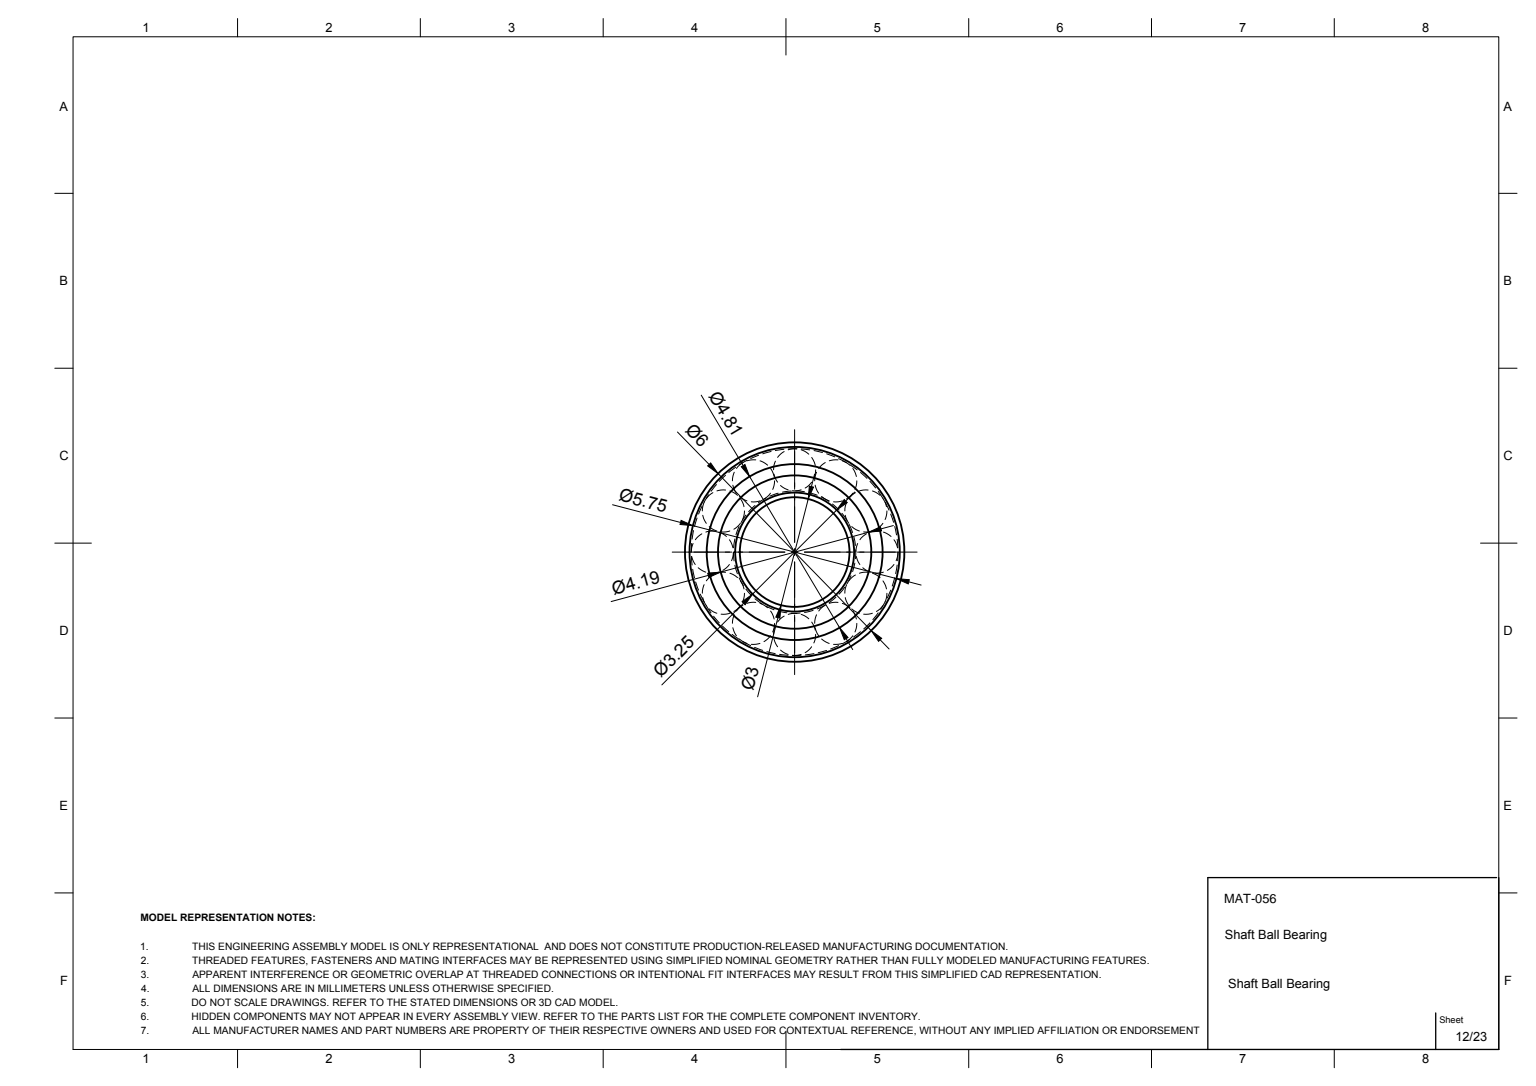
ISO-10303-21;
HEADER;
/* Generated by software containing ST-Developer
 * from STEP Tools, Inc. (www.steptools.com) 
 */

FILE_DESCRIPTION(
/* description */ (''),
/* implementation_level */ '2;1');

FILE_NAME(
/* name */ 'Shaft Ball Bearing.step',
/* time_stamp */ '2026-10-28T16:47:13+01:00',
/* author */ (''),
/* organization */ (''),
/* preprocessor_version */ 'ST-DEVELOPER v20.2',
/* originating_system */ 'Autodesk Translation Framework v15.17.0.0',
/* authorisation */ '');

FILE_SCHEMA (('AUTOMOTIVE_DESIGN { 1 0 10303 214 3 1 1 }'));
ENDSEC;

DATA;
#10=MECHANICAL_DESIGN_GEOMETRIC_PRESENTATION_REPRESENTATION('',(#4589,#4590,#4591,#4592,#4593,#4594,#4595,#4596,#4597,#4598,#4599,#4600,#4601,#4602,#4603,#4604),#459242);
#143=SPHERICAL_SURFACE('',#99208,0.576463888168111);
#144=SPHERICAL_SURFACE('',#99210,0.576463888168111);
#145=SPHERICAL_SURFACE('',#99212,0.576463888168111);
#146=SPHERICAL_SURFACE('',#99214,0.576463888168111);
#147=SPHERICAL_SURFACE('',#99216,0.576463888168111);
#148=SPHERICAL_SURFACE('',#99218,0.576463888168111);
#149=SPHERICAL_SURFACE('',#99220,0.576463888168111);
#150=SPHERICAL_SURFACE('',#99222,0.576463888168111);
#151=SPHERICAL_SURFACE('',#99224,0.576463888168111);
#152=SPHERICAL_SURFACE('',#99226,0.576463888168111);
#153=SPHERICAL_SURFACE('',#99228,0.576463888168111);
#154=SPHERICAL_SURFACE('',#99230,0.576463888168111);
#1862=TOROIDAL_SURFACE('',#99175,2.25,0.576463888168111);
#1863=TOROIDAL_SURFACE('',#99190,2.25,0.57646388816811);
#4416=SHAPE_REPRESENTATION_RELATIONSHIP('SRR','None',#459342,#4437);
#4437=ADVANCED_BREP_SHAPE_REPRESENTATION('',(#4469,#4470,#4471,#4472,#4473,
#4474,#4475,#4476,#4477,#4478,#4479,#4480,#4481,#4482,#4483,#4484),#459231);
#4469=MANIFOLD_SOLID_BREP('Body1',#94647);
#4470=MANIFOLD_SOLID_BREP('Body2',#94648);
#4471=MANIFOLD_SOLID_BREP('Body3',#94649);
#4472=MANIFOLD_SOLID_BREP('Body4',#94650);
#4473=MANIFOLD_SOLID_BREP('Body5',#94651);
#4474=MANIFOLD_SOLID_BREP('Body6',#94652);
#4475=MANIFOLD_SOLID_BREP('Body7',#94653);
#4476=MANIFOLD_SOLID_BREP('Body8',#94654);
#4477=MANIFOLD_SOLID_BREP('Body9',#94655);
#4478=MANIFOLD_SOLID_BREP('Body10',#94656);
#4479=MANIFOLD_SOLID_BREP('Body11',#94657);
#4480=MANIFOLD_SOLID_BREP('Body12',#94658);
#4481=MANIFOLD_SOLID_BREP('Body13',#94659);
#4482=MANIFOLD_SOLID_BREP('Body14',#94660);
#4483=MANIFOLD_SOLID_BREP('Body15',#94661);
#4484=MANIFOLD_SOLID_BREP('Body16',#94662);
#4589=STYLED_ITEM('',(#459526),#4469);
#4590=STYLED_ITEM('',(#459526),#4470);
#4591=STYLED_ITEM('',(#459526),#4471);
#4592=STYLED_ITEM('',(#459526),#4472);
#4593=STYLED_ITEM('',(#459526),#4473);
#4594=STYLED_ITEM('',(#459526),#4474);
#4595=STYLED_ITEM('',(#459526),#4475);
#4596=STYLED_ITEM('',(#459526),#4476);
#4597=STYLED_ITEM('',(#459526),#4477);
#4598=STYLED_ITEM('',(#459526),#4478);
#4599=STYLED_ITEM('',(#459526),#4479);
#4600=STYLED_ITEM('',(#459526),#4480);
#4601=STYLED_ITEM('',(#459526),#4481);
#4602=STYLED_ITEM('',(#459526),#4482);
#4603=STYLED_ITEM('',(#459526),#4483);
#4604=STYLED_ITEM('',(#459526),#4484);
#4884=CONICAL_SURFACE('',#99180,2.875,0.78539816339745);
#4885=CONICAL_SURFACE('',#99186,3.,0.785398163397449);
#4886=CONICAL_SURFACE('',#99194,1.625,0.785398163397448);
#4887=CONICAL_SURFACE('',#99200,1.5,0.785398163397449);
#5213=FACE_BOUND('',#14323,.T.);
#5214=FACE_BOUND('',#14325,.T.);
#5215=FACE_BOUND('',#14333,.T.);
#5216=FACE_BOUND('',#14335,.T.);
#5217=FACE_BOUND('',#14351,.T.);
#5218=FACE_BOUND('',#14353,.T.);
#5219=FACE_BOUND('',#14357,.T.);
#5220=FACE_BOUND('',#14359,.T.);
#5697=PLANE('',#99188);
#5698=PLANE('',#99189);
#5699=PLANE('',#99206);
#5700=PLANE('',#99207);
#5701=PLANE('',#99238);
#5702=PLANE('',#99239);
#5703=PLANE('',#99246);
#5704=PLANE('',#99247);
#8408=FACE_OUTER_BOUND('',#14316,.T.);
#8409=FACE_OUTER_BOUND('',#14317,.T.);
#8410=FACE_OUTER_BOUND('',#14318,.T.);
#8411=FACE_OUTER_BOUND('',#14319,.T.);
#8412=FACE_OUTER_BOUND('',#14320,.T.);
#8413=FACE_OUTER_BOUND('',#14321,.T.);
#8414=FACE_OUTER_BOUND('',#14322,.T.);
#8415=FACE_OUTER_BOUND('',#14324,.T.);
#8416=FACE_OUTER_BOUND('',#14326,.T.);
#8417=FACE_OUTER_BOUND('',#14327,.T.);
#8418=FACE_OUTER_BOUND('',#14328,.T.);
#8419=FACE_OUTER_BOUND('',#14329,.T.);
#8420=FACE_OUTER_BOUND('',#14330,.T.);
#8421=FACE_OUTER_BOUND('',#14331,.T.);
#8422=FACE_OUTER_BOUND('',#14332,.T.);
#8423=FACE_OUTER_BOUND('',#14334,.T.);
#8424=FACE_OUTER_BOUND('',#14336,.T.);
#8425=FACE_OUTER_BOUND('',#14337,.T.);
#8426=FACE_OUTER_BOUND('',#14338,.T.);
#8427=FACE_OUTER_BOUND('',#14339,.T.);
#8428=FACE_OUTER_BOUND('',#14340,.T.);
#8429=FACE_OUTER_BOUND('',#14341,.T.);
#8430=FACE_OUTER_BOUND('',#14342,.T.);
#8431=FACE_OUTER_BOUND('',#14343,.T.);
#8432=FACE_OUTER_BOUND('',#14344,.T.);
#8433=FACE_OUTER_BOUND('',#14345,.T.);
#8434=FACE_OUTER_BOUND('',#14346,.T.);
#8435=FACE_OUTER_BOUND('',#14347,.T.);
#8436=FACE_OUTER_BOUND('',#14348,.T.);
#8437=FACE_OUTER_BOUND('',#14349,.T.);
#8438=FACE_OUTER_BOUND('',#14350,.T.);
#8439=FACE_OUTER_BOUND('',#14352,.T.);
#8440=FACE_OUTER_BOUND('',#14354,.T.);
#8441=FACE_OUTER_BOUND('',#14355,.T.);
#8442=FACE_OUTER_BOUND('',#14356,.T.);
#8443=FACE_OUTER_BOUND('',#14358,.T.);
#14316=EDGE_LOOP('',(#69274,#69275,#69276,#69277));
#14317=EDGE_LOOP('',(#69278,#69279,#69280,#69281));
#14318=EDGE_LOOP('',(#69282,#69283,#69284,#69285));
#14319=EDGE_LOOP('',(#69286,#69287,#69288,#69289));
#14320=EDGE_LOOP('',(#69290,#69291,#69292,#69293,#69294));
#14321=EDGE_LOOP('',(#69295,#69296,#69297,#69298,#69299));
#14322=EDGE_LOOP('',(#69300));
#14323=EDGE_LOOP('',(#69301));
#14324=EDGE_LOOP('',(#69302));
#14325=EDGE_LOOP('',(#69303));
#14326=EDGE_LOOP('',(#69304,#69305,#69306,#69307));
#14327=EDGE_LOOP('',(#69308,#69309,#69310,#69311));
#14328=EDGE_LOOP('',(#69312,#69313,#69314,#69315,#69316));
#14329=EDGE_LOOP('',(#69317,#69318,#69319,#69320,#69321));
#14330=EDGE_LOOP('',(#69322,#69323,#69324,#69325));
#14331=EDGE_LOOP('',(#69326,#69327,#69328,#69329));
#14332=EDGE_LOOP('',(#69330));
#14333=EDGE_LOOP('',(#69331));
#14334=EDGE_LOOP('',(#69332));
#14335=EDGE_LOOP('',(#69333));
#14336=EDGE_LOOP('',(#69334,#69335));
#14337=EDGE_LOOP('',(#69336,#69337));
#14338=EDGE_LOOP('',(#69338,#69339));
#14339=EDGE_LOOP('',(#69340,#69341));
#14340=EDGE_LOOP('',(#69342,#69343));
#14341=EDGE_LOOP('',(#69344,#69345));
#14342=EDGE_LOOP('',(#69346,#69347));
#14343=EDGE_LOOP('',(#69348,#69349));
#14344=EDGE_LOOP('',(#69350,#69351));
#14345=EDGE_LOOP('',(#69352,#69353));
#14346=EDGE_LOOP('',(#69354,#69355));
#14347=EDGE_LOOP('',(#69356,#69357));
#14348=EDGE_LOOP('',(#69358,#69359,#69360,#69361));
#14349=EDGE_LOOP('',(#69362,#69363,#69364,#69365));
#14350=EDGE_LOOP('',(#69366));
#14351=EDGE_LOOP('',(#69367));
#14352=EDGE_LOOP('',(#69368));
#14353=EDGE_LOOP('',(#69369));
#14354=EDGE_LOOP('',(#69370,#69371,#69372,#69373));
#14355=EDGE_LOOP('',(#69374,#69375,#69376,#69377));
#14356=EDGE_LOOP('',(#69378));
#14357=EDGE_LOOP('',(#69379));
#14358=EDGE_LOOP('',(#69380));
#14359=EDGE_LOOP('',(#69381));
#20534=CIRCLE('',#99173,2.40384615384615);
#20535=CIRCLE('',#99174,2.40384615384615);
#20536=CIRCLE('',#99176,2.40384615384615);
#20537=CIRCLE('',#99177,0.576463888168111);
#20538=CIRCLE('',#99179,2.40384615384615);
#20539=CIRCLE('',#99181,3.);
#20540=CIRCLE('',#99182,2.875);
#20541=CIRCLE('',#99184,3.);
#20542=CIRCLE('',#99185,3.);
#20543=CIRCLE('',#99187,2.875);
#20544=CIRCLE('',#99191,2.09615384615385);
#20545=CIRCLE('',#99192,0.57646388816811);
#20546=CIRCLE('',#99193,2.09615384615385);
#20547=CIRCLE('',#99195,1.5);
#20548=CIRCLE('',#99196,1.625);
#20549=CIRCLE('',#99198,1.5);
#20550=CIRCLE('',#99199,1.5);
#20551=CIRCLE('',#99201,1.625);
#20552=CIRCLE('',#99203,2.09615384615385);
#20553=CIRCLE('',#99205,2.09615384615385);
#20554=CIRCLE('',#99209,0.576463888168111);
#20555=CIRCLE('',#99211,0.576463888168111);
#20556=CIRCLE('',#99213,0.576463888168111);
#20557=CIRCLE('',#99215,0.576463888168111);
#20558=CIRCLE('',#99217,0.576463888168111);
#20559=CIRCLE('',#99219,0.576463888168111);
#20560=CIRCLE('',#99221,0.576463888168111);
#20561=CIRCLE('',#99223,0.576463888168111);
#20562=CIRCLE('',#99225,0.576463888168111);
#20563=CIRCLE('',#99227,0.576463888168111);
#20564=CIRCLE('',#99229,0.576463888168111);
#20565=CIRCLE('',#99231,0.576463888168111);
#20566=CIRCLE('',#99233,2.40384615384615);
#20567=CIRCLE('',#99234,2.40384615384615);
#20568=CIRCLE('',#99236,2.09615384615385);
#20569=CIRCLE('',#99237,2.09615384615385);
#20570=CIRCLE('',#99241,2.40384615384615);
#20571=CIRCLE('',#99242,2.40384615384615);
#20572=CIRCLE('',#99244,2.09615384615385);
#20573=CIRCLE('',#99245,2.09615384615385);
#28975=LINE('',#366189,#32777);
#28976=LINE('',#366198,#32778);
#28977=LINE('',#366203,#32779);
#28978=LINE('',#366210,#32780);
#28979=LINE('',#366213,#32781);
#28980=LINE('',#366227,#32782);
#28981=LINE('',#366234,#32783);
#28982=LINE('',#366237,#32784);
#28983=LINE('',#366241,#32785);
#28984=LINE('',#366246,#32786);
#28985=LINE('',#366301,#32787);
#28986=LINE('',#366307,#32788);
#28987=LINE('',#366315,#32789);
#28988=LINE('',#366321,#32790);
#32777=VECTOR('',#116043,2.40384615384615);
#32778=VECTOR('',#116056,2.40384615384615);
#32779=VECTOR('',#116061,2.875);
#32780=VECTOR('',#116070,3.);
#32781=VECTOR('',#116073,3.);
#32782=VECTOR('',#116092,1.625);
#32783=VECTOR('',#116101,1.5);
#32784=VECTOR('',#116104,1.5);
#32785=VECTOR('',#116109,2.09615384615385);
#32786=VECTOR('',#116116,2.09615384615385);
#32787=VECTOR('',#116173,2.40384615384615);
#32788=VECTOR('',#116180,2.09615384615385);
#32789=VECTOR('',#116191,2.40384615384615);
#32790=VECTOR('',#116198,2.09615384615385);
#38293=VERTEX_POINT('',#366186);
#38294=VERTEX_POINT('',#366188);
#38295=VERTEX_POINT('',#366192);
#38296=VERTEX_POINT('',#366196);
#38297=VERTEX_POINT('',#366200);
#38298=VERTEX_POINT('',#366202);
#38299=VERTEX_POINT('',#366206);
#38300=VERTEX_POINT('',#366207);
#38301=VERTEX_POINT('',#366212);
#38302=VERTEX_POINT('',#366218);
#38303=VERTEX_POINT('',#366220);
#38304=VERTEX_POINT('',#366224);
#38305=VERTEX_POINT('',#366226);
#38306=VERTEX_POINT('',#366230);
#38307=VERTEX_POINT('',#366231);
#38308=VERTEX_POINT('',#366236);
#38309=VERTEX_POINT('',#366240);
#38310=VERTEX_POINT('',#366244);
#38311=VERTEX_POINT('',#366250);
#38312=VERTEX_POINT('',#366251);
#38313=VERTEX_POINT('',#366254);
#38314=VERTEX_POINT('',#366255);
#38315=VERTEX_POINT('',#366258);
#38316=VERTEX_POINT('',#366259);
#38317=VERTEX_POINT('',#366262);
#38318=VERTEX_POINT('',#366263);
#38319=VERTEX_POINT('',#366266);
#38320=VERTEX_POINT('',#366267);
#38321=VERTEX_POINT('',#366270);
#38322=VERTEX_POINT('',#366271);
#38323=VERTEX_POINT('',#366274);
#38324=VERTEX_POINT('',#366275);
#38325=VERTEX_POINT('',#366278);
#38326=VERTEX_POINT('',#366279);
#38327=VERTEX_POINT('',#366282);
#38328=VERTEX_POINT('',#366283);
#38329=VERTEX_POINT('',#366286);
#38330=VERTEX_POINT('',#366287);
#38331=VERTEX_POINT('',#366290);
#38332=VERTEX_POINT('',#366291);
#38333=VERTEX_POINT('',#366294);
#38334=VERTEX_POINT('',#366295);
#38335=VERTEX_POINT('',#366298);
#38336=VERTEX_POINT('',#366300);
#38337=VERTEX_POINT('',#366304);
#38338=VERTEX_POINT('',#366306);
#38339=VERTEX_POINT('',#366312);
#38340=VERTEX_POINT('',#366314);
#38341=VERTEX_POINT('',#366318);
#38342=VERTEX_POINT('',#366320);
#49139=EDGE_CURVE('',#38293,#38293,#20534,.T.);
#49140=EDGE_CURVE('',#38293,#38294,#28975,.T.);
#49141=EDGE_CURVE('',#38294,#38294,#20535,.T.);
#49142=EDGE_CURVE('',#38295,#38295,#20536,.T.);
#49143=EDGE_CURVE('',#38295,#38293,#20537,.T.);
#49144=EDGE_CURVE('',#38296,#38296,#20538,.T.);
#49145=EDGE_CURVE('',#38296,#38295,#28976,.T.);
#49146=EDGE_CURVE('',#38297,#38297,#20539,.T.);
#49147=EDGE_CURVE('',#38297,#38298,#28977,.T.);
#49148=EDGE_CURVE('',#38298,#38298,#20540,.T.);
#49149=EDGE_CURVE('',#38299,#38300,#20541,.T.);
#49150=EDGE_CURVE('',#38300,#38299,#20542,.T.);
#49151=EDGE_CURVE('',#38300,#38297,#28978,.T.);
#49152=EDGE_CURVE('',#38299,#38301,#28979,.T.);
#49153=EDGE_CURVE('',#38301,#38301,#20543,.T.);
#49154=EDGE_CURVE('',#38302,#38302,#20544,.T.);
#49155=EDGE_CURVE('',#38302,#38303,#20545,.T.);
#49156=EDGE_CURVE('',#38303,#38303,#20546,.T.);
#49157=EDGE_CURVE('',#38304,#38304,#20547,.T.);
#49158=EDGE_CURVE('',#38304,#38305,#28980,.T.);
#49159=EDGE_CURVE('',#38305,#38305,#20548,.T.);
#49160=EDGE_CURVE('',#38306,#38307,#20549,.T.);
#49161=EDGE_CURVE('',#38307,#38306,#20550,.T.);
#49162=EDGE_CURVE('',#38307,#38304,#28981,.T.);
#49163=EDGE_CURVE('',#38306,#38308,#28982,.T.);
#49164=EDGE_CURVE('',#38308,#38308,#20551,.T.);
#49165=EDGE_CURVE('',#38303,#38309,#28983,.T.);
#49166=EDGE_CURVE('',#38309,#38309,#20552,.T.);
#49167=EDGE_CURVE('',#38310,#38310,#20553,.T.);
#49168=EDGE_CURVE('',#38310,#38302,#28984,.T.);
#49169=EDGE_CURVE('',#38311,#38312,#20554,.T.);
#49170=EDGE_CURVE('',#38313,#38314,#20555,.T.);
#49171=EDGE_CURVE('',#38315,#38316,#20556,.T.);
#49172=EDGE_CURVE('',#38317,#38318,#20557,.T.);
#49173=EDGE_CURVE('',#38319,#38320,#20558,.T.);
#49174=EDGE_CURVE('',#38321,#38322,#20559,.T.);
#49175=EDGE_CURVE('',#38323,#38324,#20560,.T.);
#49176=EDGE_CURVE('',#38325,#38326,#20561,.T.);
#49177=EDGE_CURVE('',#38327,#38328,#20562,.T.);
#49178=EDGE_CURVE('',#38329,#38330,#20563,.T.);
#49179=EDGE_CURVE('',#38331,#38332,#20564,.T.);
#49180=EDGE_CURVE('',#38333,#38334,#20565,.T.);
#49181=EDGE_CURVE('',#38335,#38335,#20566,.T.);
#49182=EDGE_CURVE('',#38335,#38336,#28985,.T.);
#49183=EDGE_CURVE('',#38336,#38336,#20567,.T.);
#49184=EDGE_CURVE('',#38337,#38337,#20568,.T.);
#49185=EDGE_CURVE('',#38337,#38338,#28986,.T.);
#49186=EDGE_CURVE('',#38338,#38338,#20569,.T.);
#49187=EDGE_CURVE('',#38339,#38339,#20570,.T.);
#49188=EDGE_CURVE('',#38339,#38340,#28987,.T.);
#49189=EDGE_CURVE('',#38340,#38340,#20571,.T.);
#49190=EDGE_CURVE('',#38341,#38341,#20572,.T.);
#49191=EDGE_CURVE('',#38341,#38342,#28988,.T.);
#49192=EDGE_CURVE('',#38342,#38342,#20573,.T.);
#69274=ORIENTED_EDGE('',*,*,#49139,.F.);
#69275=ORIENTED_EDGE('',*,*,#49140,.T.);
#69276=ORIENTED_EDGE('',*,*,#49141,.T.);
#69277=ORIENTED_EDGE('',*,*,#49140,.F.);
#69278=ORIENTED_EDGE('',*,*,#49142,.F.);
#69279=ORIENTED_EDGE('',*,*,#49143,.T.);
#69280=ORIENTED_EDGE('',*,*,#49139,.T.);
#69281=ORIENTED_EDGE('',*,*,#49143,.F.);
#69282=ORIENTED_EDGE('',*,*,#49144,.F.);
#69283=ORIENTED_EDGE('',*,*,#49145,.T.);
#69284=ORIENTED_EDGE('',*,*,#49142,.T.);
#69285=ORIENTED_EDGE('',*,*,#49145,.F.);
#69286=ORIENTED_EDGE('',*,*,#49146,.F.);
#69287=ORIENTED_EDGE('',*,*,#49147,.T.);
#69288=ORIENTED_EDGE('',*,*,#49148,.T.);
#69289=ORIENTED_EDGE('',*,*,#49147,.F.);
#69290=ORIENTED_EDGE('',*,*,#49149,.F.);
#69291=ORIENTED_EDGE('',*,*,#49150,.F.);
#69292=ORIENTED_EDGE('',*,*,#49151,.T.);
#69293=ORIENTED_EDGE('',*,*,#49146,.T.);
#69294=ORIENTED_EDGE('',*,*,#49151,.F.);
#69295=ORIENTED_EDGE('',*,*,#49149,.T.);
#69296=ORIENTED_EDGE('',*,*,#49150,.T.);
#69297=ORIENTED_EDGE('',*,*,#49152,.T.);
#69298=ORIENTED_EDGE('',*,*,#49153,.F.);
#69299=ORIENTED_EDGE('',*,*,#49152,.F.);
#69300=ORIENTED_EDGE('',*,*,#49148,.F.);
#69301=ORIENTED_EDGE('',*,*,#49144,.T.);
#69302=ORIENTED_EDGE('',*,*,#49153,.T.);
#69303=ORIENTED_EDGE('',*,*,#49141,.F.);
#69304=ORIENTED_EDGE('',*,*,#49154,.F.);
#69305=ORIENTED_EDGE('',*,*,#49155,.T.);
#69306=ORIENTED_EDGE('',*,*,#49156,.T.);
#69307=ORIENTED_EDGE('',*,*,#49155,.F.);
#69308=ORIENTED_EDGE('',*,*,#49157,.F.);
#69309=ORIENTED_EDGE('',*,*,#49158,.T.);
#69310=ORIENTED_EDGE('',*,*,#49159,.T.);
#69311=ORIENTED_EDGE('',*,*,#49158,.F.);
#69312=ORIENTED_EDGE('',*,*,#49160,.F.);
#69313=ORIENTED_EDGE('',*,*,#49161,.F.);
#69314=ORIENTED_EDGE('',*,*,#49162,.T.);
#69315=ORIENTED_EDGE('',*,*,#49157,.T.);
#69316=ORIENTED_EDGE('',*,*,#49162,.F.);
#69317=ORIENTED_EDGE('',*,*,#49160,.T.);
#69318=ORIENTED_EDGE('',*,*,#49161,.T.);
#69319=ORIENTED_EDGE('',*,*,#49163,.T.);
#69320=ORIENTED_EDGE('',*,*,#49164,.F.);
#69321=ORIENTED_EDGE('',*,*,#49163,.F.);
#69322=ORIENTED_EDGE('',*,*,#49156,.F.);
#69323=ORIENTED_EDGE('',*,*,#49165,.T.);
#69324=ORIENTED_EDGE('',*,*,#49166,.T.);
#69325=ORIENTED_EDGE('',*,*,#49165,.F.);
#69326=ORIENTED_EDGE('',*,*,#49167,.F.);
#69327=ORIENTED_EDGE('',*,*,#49168,.T.);
#69328=ORIENTED_EDGE('',*,*,#49154,.T.);
#69329=ORIENTED_EDGE('',*,*,#49168,.F.);
#69330=ORIENTED_EDGE('',*,*,#49167,.T.);
#69331=ORIENTED_EDGE('',*,*,#49159,.F.);
#69332=ORIENTED_EDGE('',*,*,#49166,.F.);
#69333=ORIENTED_EDGE('',*,*,#49164,.T.);
#69334=ORIENTED_EDGE('',*,*,#49169,.T.);
#69335=ORIENTED_EDGE('',*,*,#49169,.F.);
#69336=ORIENTED_EDGE('',*,*,#49170,.T.);
#69337=ORIENTED_EDGE('',*,*,#49170,.F.);
#69338=ORIENTED_EDGE('',*,*,#49171,.T.);
#69339=ORIENTED_EDGE('',*,*,#49171,.F.);
#69340=ORIENTED_EDGE('',*,*,#49172,.T.);
#69341=ORIENTED_EDGE('',*,*,#49172,.F.);
#69342=ORIENTED_EDGE('',*,*,#49173,.T.);
#69343=ORIENTED_EDGE('',*,*,#49173,.F.);
#69344=ORIENTED_EDGE('',*,*,#49174,.T.);
#69345=ORIENTED_EDGE('',*,*,#49174,.F.);
#69346=ORIENTED_EDGE('',*,*,#49175,.T.);
#69347=ORIENTED_EDGE('',*,*,#49175,.F.);
#69348=ORIENTED_EDGE('',*,*,#49176,.T.);
#69349=ORIENTED_EDGE('',*,*,#49176,.F.);
#69350=ORIENTED_EDGE('',*,*,#49177,.T.);
#69351=ORIENTED_EDGE('',*,*,#49177,.F.);
#69352=ORIENTED_EDGE('',*,*,#49178,.T.);
#69353=ORIENTED_EDGE('',*,*,#49178,.F.);
#69354=ORIENTED_EDGE('',*,*,#49179,.T.);
#69355=ORIENTED_EDGE('',*,*,#49179,.F.);
#69356=ORIENTED_EDGE('',*,*,#49180,.T.);
#69357=ORIENTED_EDGE('',*,*,#49180,.F.);
#69358=ORIENTED_EDGE('',*,*,#49181,.F.);
#69359=ORIENTED_EDGE('',*,*,#49182,.T.);
#69360=ORIENTED_EDGE('',*,*,#49183,.T.);
#69361=ORIENTED_EDGE('',*,*,#49182,.F.);
#69362=ORIENTED_EDGE('',*,*,#49184,.F.);
#69363=ORIENTED_EDGE('',*,*,#49185,.T.);
#69364=ORIENTED_EDGE('',*,*,#49186,.T.);
#69365=ORIENTED_EDGE('',*,*,#49185,.F.);
#69366=ORIENTED_EDGE('',*,*,#49181,.T.);
#69367=ORIENTED_EDGE('',*,*,#49186,.F.);
#69368=ORIENTED_EDGE('',*,*,#49183,.F.);
#69369=ORIENTED_EDGE('',*,*,#49184,.T.);
#69370=ORIENTED_EDGE('',*,*,#49187,.F.);
#69371=ORIENTED_EDGE('',*,*,#49188,.T.);
#69372=ORIENTED_EDGE('',*,*,#49189,.T.);
#69373=ORIENTED_EDGE('',*,*,#49188,.F.);
#69374=ORIENTED_EDGE('',*,*,#49190,.F.);
#69375=ORIENTED_EDGE('',*,*,#49191,.T.);
#69376=ORIENTED_EDGE('',*,*,#49192,.T.);
#69377=ORIENTED_EDGE('',*,*,#49191,.F.);
#69378=ORIENTED_EDGE('',*,*,#49189,.F.);
#69379=ORIENTED_EDGE('',*,*,#49190,.T.);
#69380=ORIENTED_EDGE('',*,*,#49187,.T.);
#69381=ORIENTED_EDGE('',*,*,#49192,.F.);
#87921=CYLINDRICAL_SURFACE('',#99172,2.40384615384615);
#87922=CYLINDRICAL_SURFACE('',#99178,2.40384615384615);
#87923=CYLINDRICAL_SURFACE('',#99183,3.);
#87924=CYLINDRICAL_SURFACE('',#99197,1.5);
#87925=CYLINDRICAL_SURFACE('',#99202,2.09615384615385);
#87926=CYLINDRICAL_SURFACE('',#99204,2.09615384615385);
#87927=CYLINDRICAL_SURFACE('',#99232,2.40384615384615);
#87928=CYLINDRICAL_SURFACE('',#99235,2.09615384615385);
#87929=CYLINDRICAL_SURFACE('',#99240,2.40384615384615);
#87930=CYLINDRICAL_SURFACE('',#99243,2.09615384615385);
#90872=ADVANCED_FACE('',(#8408),#87921,.F.);
#90873=ADVANCED_FACE('',(#8409),#1862,.F.);
#90874=ADVANCED_FACE('',(#8410),#87922,.F.);
#90875=ADVANCED_FACE('',(#8411),#4884,.T.);
#90876=ADVANCED_FACE('',(#8412),#87923,.T.);
#90877=ADVANCED_FACE('',(#8413),#4885,.T.);
#90878=ADVANCED_FACE('',(#8414,#5213),#5697,.F.);
#90879=ADVANCED_FACE('',(#8415,#5214),#5698,.F.);
#90880=ADVANCED_FACE('',(#8416),#1863,.F.);
#90881=ADVANCED_FACE('',(#8417),#4886,.F.);
#90882=ADVANCED_FACE('',(#8418),#87924,.F.);
#90883=ADVANCED_FACE('',(#8419),#4887,.F.);
#90884=ADVANCED_FACE('',(#8420),#87925,.T.);
#90885=ADVANCED_FACE('',(#8421),#87926,.T.);
#90886=ADVANCED_FACE('',(#8422,#5215),#5699,.F.);
#90887=ADVANCED_FACE('',(#8423,#5216),#5700,.F.);
#90888=ADVANCED_FACE('',(#8424),#143,.T.);
#90889=ADVANCED_FACE('',(#8425),#144,.T.);
#90890=ADVANCED_FACE('',(#8426),#145,.T.);
#90891=ADVANCED_FACE('',(#8427),#146,.T.);
#90892=ADVANCED_FACE('',(#8428),#147,.T.);
#90893=ADVANCED_FACE('',(#8429),#148,.T.);
#90894=ADVANCED_FACE('',(#8430),#149,.T.);
#90895=ADVANCED_FACE('',(#8431),#150,.T.);
#90896=ADVANCED_FACE('',(#8432),#151,.T.);
#90897=ADVANCED_FACE('',(#8433),#152,.T.);
#90898=ADVANCED_FACE('',(#8434),#153,.T.);
#90899=ADVANCED_FACE('',(#8435),#154,.T.);
#90900=ADVANCED_FACE('',(#8436),#87927,.T.);
#90901=ADVANCED_FACE('',(#8437),#87928,.F.);
#90902=ADVANCED_FACE('',(#8438,#5217),#5701,.F.);
#90903=ADVANCED_FACE('',(#8439,#5218),#5702,.F.);
#90904=ADVANCED_FACE('',(#8440),#87929,.T.);
#90905=ADVANCED_FACE('',(#8441),#87930,.F.);
#90906=ADVANCED_FACE('',(#8442,#5219),#5703,.F.);
#90907=ADVANCED_FACE('',(#8443,#5220),#5704,.F.);
#94647=CLOSED_SHELL('',(#90872,#90873,#90874,#90875,#90876,#90877,#90878,
#90879));
#94648=CLOSED_SHELL('',(#90880,#90881,#90882,#90883,#90884,#90885,#90886,
#90887));
#94649=CLOSED_SHELL('',(#90888));
#94650=CLOSED_SHELL('',(#90889));
#94651=CLOSED_SHELL('',(#90890));
#94652=CLOSED_SHELL('',(#90891));
#94653=CLOSED_SHELL('',(#90892));
#94654=CLOSED_SHELL('',(#90893));
#94655=CLOSED_SHELL('',(#90894));
#94656=CLOSED_SHELL('',(#90895));
#94657=CLOSED_SHELL('',(#90896));
#94658=CLOSED_SHELL('',(#90897));
#94659=CLOSED_SHELL('',(#90898));
#94660=CLOSED_SHELL('',(#90899));
#94661=CLOSED_SHELL('',(#90900,#90901,#90902,#90903));
#94662=CLOSED_SHELL('',(#90904,#90905,#90906,#90907));
#99171=AXIS2_PLACEMENT_3D('',#366184,#116037,#116038);
#99172=AXIS2_PLACEMENT_3D('',#366185,#116039,#116040);
#99173=AXIS2_PLACEMENT_3D('',#366187,#116041,#116042);
#99174=AXIS2_PLACEMENT_3D('',#366190,#116044,#116045);
#99175=AXIS2_PLACEMENT_3D('',#366191,#116046,#116047);
#99176=AXIS2_PLACEMENT_3D('',#366193,#116048,#116049);
#99177=AXIS2_PLACEMENT_3D('',#366194,#116050,#116051);
#99178=AXIS2_PLACEMENT_3D('',#366195,#116052,#116053);
#99179=AXIS2_PLACEMENT_3D('',#366197,#116054,#116055);
#99180=AXIS2_PLACEMENT_3D('',#366199,#116057,#116058);
#99181=AXIS2_PLACEMENT_3D('',#366201,#116059,#116060);
#99182=AXIS2_PLACEMENT_3D('',#366204,#116062,#116063);
#99183=AXIS2_PLACEMENT_3D('',#366205,#116064,#116065);
#99184=AXIS2_PLACEMENT_3D('',#366208,#116066,#116067);
#99185=AXIS2_PLACEMENT_3D('',#366209,#116068,#116069);
#99186=AXIS2_PLACEMENT_3D('',#366211,#116071,#116072);
#99187=AXIS2_PLACEMENT_3D('',#366214,#116074,#116075);
#99188=AXIS2_PLACEMENT_3D('',#366215,#116076,#116077);
#99189=AXIS2_PLACEMENT_3D('',#366216,#116078,#116079);
#99190=AXIS2_PLACEMENT_3D('',#366217,#116080,#116081);
#99191=AXIS2_PLACEMENT_3D('',#366219,#116082,#116083);
#99192=AXIS2_PLACEMENT_3D('',#366221,#116084,#116085);
#99193=AXIS2_PLACEMENT_3D('',#366222,#116086,#116087);
#99194=AXIS2_PLACEMENT_3D('',#366223,#116088,#116089);
#99195=AXIS2_PLACEMENT_3D('',#366225,#116090,#116091);
#99196=AXIS2_PLACEMENT_3D('',#366228,#116093,#116094);
#99197=AXIS2_PLACEMENT_3D('',#366229,#116095,#116096);
#99198=AXIS2_PLACEMENT_3D('',#366232,#116097,#116098);
#99199=AXIS2_PLACEMENT_3D('',#366233,#116099,#116100);
#99200=AXIS2_PLACEMENT_3D('',#366235,#116102,#116103);
#99201=AXIS2_PLACEMENT_3D('',#366238,#116105,#116106);
#99202=AXIS2_PLACEMENT_3D('',#366239,#116107,#116108);
#99203=AXIS2_PLACEMENT_3D('',#366242,#116110,#116111);
#99204=AXIS2_PLACEMENT_3D('',#366243,#116112,#116113);
#99205=AXIS2_PLACEMENT_3D('',#366245,#116114,#116115);
#99206=AXIS2_PLACEMENT_3D('',#366247,#116117,#116118);
#99207=AXIS2_PLACEMENT_3D('',#366248,#116119,#116120);
#99208=AXIS2_PLACEMENT_3D('',#366249,#116121,#116122);
#99209=AXIS2_PLACEMENT_3D('',#366252,#116123,#116124);
#99210=AXIS2_PLACEMENT_3D('',#366253,#116125,#116126);
#99211=AXIS2_PLACEMENT_3D('',#366256,#116127,#116128);
#99212=AXIS2_PLACEMENT_3D('',#366257,#116129,#116130);
#99213=AXIS2_PLACEMENT_3D('',#366260,#116131,#116132);
#99214=AXIS2_PLACEMENT_3D('',#366261,#116133,#116134);
#99215=AXIS2_PLACEMENT_3D('',#366264,#116135,#116136);
#99216=AXIS2_PLACEMENT_3D('',#366265,#116137,#116138);
#99217=AXIS2_PLACEMENT_3D('',#366268,#116139,#116140);
#99218=AXIS2_PLACEMENT_3D('',#366269,#116141,#116142);
#99219=AXIS2_PLACEMENT_3D('',#366272,#116143,#116144);
#99220=AXIS2_PLACEMENT_3D('',#366273,#116145,#116146);
#99221=AXIS2_PLACEMENT_3D('',#366276,#116147,#116148);
#99222=AXIS2_PLACEMENT_3D('',#366277,#116149,#116150);
#99223=AXIS2_PLACEMENT_3D('',#366280,#116151,#116152);
#99224=AXIS2_PLACEMENT_3D('',#366281,#116153,#116154);
#99225=AXIS2_PLACEMENT_3D('',#366284,#116155,#116156);
#99226=AXIS2_PLACEMENT_3D('',#366285,#116157,#116158);
#99227=AXIS2_PLACEMENT_3D('',#366288,#116159,#116160);
#99228=AXIS2_PLACEMENT_3D('',#366289,#116161,#116162);
#99229=AXIS2_PLACEMENT_3D('',#366292,#116163,#116164);
#99230=AXIS2_PLACEMENT_3D('',#366293,#116165,#116166);
#99231=AXIS2_PLACEMENT_3D('',#366296,#116167,#116168);
#99232=AXIS2_PLACEMENT_3D('',#366297,#116169,#116170);
#99233=AXIS2_PLACEMENT_3D('',#366299,#116171,#116172);
#99234=AXIS2_PLACEMENT_3D('',#366302,#116174,#116175);
#99235=AXIS2_PLACEMENT_3D('',#366303,#116176,#116177);
#99236=AXIS2_PLACEMENT_3D('',#366305,#116178,#116179);
#99237=AXIS2_PLACEMENT_3D('',#366308,#116181,#116182);
#99238=AXIS2_PLACEMENT_3D('',#366309,#116183,#116184);
#99239=AXIS2_PLACEMENT_3D('',#366310,#116185,#116186);
#99240=AXIS2_PLACEMENT_3D('',#366311,#116187,#116188);
#99241=AXIS2_PLACEMENT_3D('',#366313,#116189,#116190);
#99242=AXIS2_PLACEMENT_3D('',#366316,#116192,#116193);
#99243=AXIS2_PLACEMENT_3D('',#366317,#116194,#116195);
#99244=AXIS2_PLACEMENT_3D('',#366319,#116196,#116197);
#99245=AXIS2_PLACEMENT_3D('',#366322,#116199,#116200);
#99246=AXIS2_PLACEMENT_3D('',#366323,#116201,#116202);
#99247=AXIS2_PLACEMENT_3D('',#366324,#116203,#116204);
#116037=DIRECTION('axis',(0.,0.,1.));
#116038=DIRECTION('refdir',(1.,0.,0.));
#116039=DIRECTION('center_axis',(0.,0.,1.));
#116040=DIRECTION('ref_axis',(1.,0.,0.));
#116041=DIRECTION('center_axis',(0.,0.,1.));
#116042=DIRECTION('ref_axis',(1.,0.,0.));
#116043=DIRECTION('',(0.,0.,1.));
#116044=DIRECTION('center_axis',(0.,0.,1.));
#116045=DIRECTION('ref_axis',(1.,0.,0.));
#116046=DIRECTION('center_axis',(0.,0.,1.));
#116047=DIRECTION('ref_axis',(1.,0.,0.));
#116048=DIRECTION('center_axis',(0.,0.,1.));
#116049=DIRECTION('ref_axis',(1.,0.,0.));
#116050=DIRECTION('center_axis',(-1.22464679914735E-16,1.,0.));
#116051=DIRECTION('ref_axis',(-1.,-1.22464679914735E-16,0.));
#116052=DIRECTION('center_axis',(0.,0.,1.));
#116053=DIRECTION('ref_axis',(1.,0.,0.));
#116054=DIRECTION('center_axis',(0.,0.,1.));
#116055=DIRECTION('ref_axis',(1.,0.,0.));
#116056=DIRECTION('',(0.,0.,1.));
#116057=DIRECTION('center_axis',(0.,0.,1.));
#116058=DIRECTION('ref_axis',(1.,0.,0.));
#116059=DIRECTION('center_axis',(0.,0.,1.));
#116060=DIRECTION('ref_axis',(1.,0.,0.));
#116061=DIRECTION('',(0.707106781186549,8.65956056235495E-17,-0.707106781186546));
#116062=DIRECTION('center_axis',(0.,0.,1.));
#116063=DIRECTION('ref_axis',(1.,0.,0.));
#116064=DIRECTION('center_axis',(0.,0.,1.));
#116065=DIRECTION('ref_axis',(1.,0.,0.));
#116066=DIRECTION('center_axis',(0.,0.,1.));
#116067=DIRECTION('ref_axis',(1.,0.,0.));
#116068=DIRECTION('center_axis',(0.,0.,1.));
#116069=DIRECTION('ref_axis',(1.,0.,0.));
#116070=DIRECTION('',(0.,0.,-1.));
#116071=DIRECTION('center_axis',(0.,0.,-1.));
#116072=DIRECTION('ref_axis',(-1.,0.,0.));
#116073=DIRECTION('',(-0.707106781186548,8.65956056235494E-17,0.707106781186547));
#116074=DIRECTION('center_axis',(0.,0.,1.));
#116075=DIRECTION('ref_axis',(1.,0.,0.));
#116076=DIRECTION('center_axis',(0.,0.,1.));
#116077=DIRECTION('ref_axis',(1.,0.,0.));
#116078=DIRECTION('center_axis',(0.,0.,-1.));
#116079=DIRECTION('ref_axis',(-1.,0.,0.));
#116080=DIRECTION('center_axis',(0.,0.,1.));
#116081=DIRECTION('ref_axis',(1.,0.,0.));
#116082=DIRECTION('center_axis',(0.,0.,1.));
#116083=DIRECTION('ref_axis',(1.,0.,0.));
#116084=DIRECTION('center_axis',(-1.22464679914735E-16,1.,0.));
#116085=DIRECTION('ref_axis',(-1.,-1.22464679914735E-16,0.));
#116086=DIRECTION('center_axis',(0.,0.,1.));
#116087=DIRECTION('ref_axis',(1.,0.,0.));
#116088=DIRECTION('center_axis',(0.,0.,1.));
#116089=DIRECTION('ref_axis',(1.,0.,0.));
#116090=DIRECTION('center_axis',(0.,0.,1.));
#116091=DIRECTION('ref_axis',(1.,0.,0.));
#116092=DIRECTION('',(-0.707106781186547,-8.65956056235493E-17,0.707106781186548));
#116093=DIRECTION('center_axis',(0.,0.,1.));
#116094=DIRECTION('ref_axis',(1.,0.,0.));
#116095=DIRECTION('center_axis',(0.,0.,1.));
#116096=DIRECTION('ref_axis',(1.,0.,0.));
#116097=DIRECTION('center_axis',(0.,0.,1.));
#116098=DIRECTION('ref_axis',(1.,0.,0.));
#116099=DIRECTION('center_axis',(0.,0.,1.));
#116100=DIRECTION('ref_axis',(1.,0.,0.));
#116101=DIRECTION('',(0.,0.,1.));
#116102=DIRECTION('center_axis',(0.,0.,-1.));
#116103=DIRECTION('ref_axis',(-1.,0.,0.));
#116104=DIRECTION('',(0.707106781186548,-8.65956056235494E-17,-0.707106781186547));
#116105=DIRECTION('center_axis',(0.,0.,1.));
#116106=DIRECTION('ref_axis',(1.,0.,0.));
#116107=DIRECTION('center_axis',(0.,0.,1.));
#116108=DIRECTION('ref_axis',(1.,0.,0.));
#116109=DIRECTION('',(0.,0.,-1.));
#116110=DIRECTION('center_axis',(0.,0.,1.));
#116111=DIRECTION('ref_axis',(1.,0.,0.));
#116112=DIRECTION('center_axis',(0.,0.,1.));
#116113=DIRECTION('ref_axis',(1.,0.,0.));
#116114=DIRECTION('center_axis',(0.,0.,1.));
#116115=DIRECTION('ref_axis',(1.,0.,0.));
#116116=DIRECTION('',(0.,0.,-1.));
#116117=DIRECTION('center_axis',(0.,0.,-1.));
#116118=DIRECTION('ref_axis',(-1.,0.,0.));
#116119=DIRECTION('center_axis',(0.,0.,1.));
#116120=DIRECTION('ref_axis',(1.,0.,0.));
#116121=DIRECTION('center_axis',(-1.,0.,0.));
#116122=DIRECTION('ref_axis',(0.,1.,0.));
#116123=DIRECTION('center_axis',(0.,1.22464679914735E-16,1.));
#116124=DIRECTION('ref_axis',(0.,-1.,1.22464679914735E-16));
#116125=DIRECTION('center_axis',(-0.866025403784438,0.500000000000001,0.));
#116126=DIRECTION('ref_axis',(0.500000000000001,0.866025403784438,0.));
#116127=DIRECTION('center_axis',(6.12323399573678E-17,1.06057523872491E-16,
1.));
#116128=DIRECTION('ref_axis',(-0.500000000000001,-0.866025403784438,1.22464679914735E-16));
#116129=DIRECTION('center_axis',(-0.499999999999998,0.86602540378444,0.));
#116130=DIRECTION('ref_axis',(0.86602540378444,0.499999999999998,0.));
#116131=DIRECTION('center_axis',(1.06057523872491E-16,6.12323399573674E-17,
1.));
#116132=DIRECTION('ref_axis',(-0.86602540378444,-0.499999999999998,1.22464679914735E-16));
#116133=DIRECTION('center_axis',(3.85183893531728E-15,1.,0.));
#116134=DIRECTION('ref_axis',(1.,-3.49148133884313E-15,0.));
#116135=DIRECTION('center_axis',(1.22464679914735E-16,-4.27583144589696E-31,
1.));
#116136=DIRECTION('ref_axis',(-1.,3.49148133884314E-15,1.22464679914735E-16));
#116137=DIRECTION('center_axis',(0.500000000000004,0.866025403784436,0.));
#116138=DIRECTION('ref_axis',(0.866025403784436,-0.500000000000004,0.));
#116139=DIRECTION('center_axis',(1.0605752387249E-16,-6.12323399573682E-17,
1.));
#116140=DIRECTION('ref_axis',(-0.866025403784436,0.500000000000004,1.22464679914735E-16));
#116141=DIRECTION('center_axis',(0.866025403784442,0.499999999999995,0.));
#116142=DIRECTION('ref_axis',(0.499999999999995,-0.866025403784442,0.));
#116143=DIRECTION('center_axis',(6.1232339957367E-17,-1.06057523872491E-16,
1.));
#116144=DIRECTION('ref_axis',(-0.499999999999995,0.866025403784442,1.22464679914735E-16));
#116145=DIRECTION('center_axis',(1.,-6.9333100835711E-15,0.));
#116146=DIRECTION('ref_axis',(-6.98296267768627E-15,-1.,0.));
#116147=DIRECTION('center_axis',(-8.55166289179392E-31,-1.22464679914735E-16,
1.));
#116148=DIRECTION('ref_axis',(6.98296267768627E-15,1.,1.22464679914735E-16));
#116149=DIRECTION('center_axis',(0.866025403784434,-0.500000000000007,0.));
#116150=DIRECTION('ref_axis',(-0.500000000000008,-0.866025403784434,0.));
#116151=DIRECTION('center_axis',(-6.12323399573685E-17,-1.0605752387249E-16,
1.));
#116152=DIRECTION('ref_axis',(0.500000000000007,0.866025403784435,1.22464679914735E-16));
#116153=DIRECTION('center_axis',(0.499999999999992,-0.866025403784443,0.));
#116154=DIRECTION('ref_axis',(-0.866025403784443,-0.499999999999992,0.));
#116155=DIRECTION('center_axis',(-1.06057523872491E-16,-6.12323399573667E-17,
1.));
#116156=DIRECTION('ref_axis',(0.866025403784443,0.499999999999992,1.22464679914735E-16));
#116157=DIRECTION('center_axis',(-1.07851490188884E-14,-1.,0.));
#116158=DIRECTION('ref_axis',(-1.,1.04744440165294E-14,0.));
#116159=DIRECTION('center_axis',(-1.22464679914735E-16,1.28274943376909E-30,
1.));
#116160=DIRECTION('ref_axis',(1.,-1.04744440165294E-14,1.22464679914735E-16));
#116161=DIRECTION('center_axis',(-0.50000000000001,-0.866025403784433,0.));
#116162=DIRECTION('ref_axis',(-0.866025403784433,0.50000000000001,0.));
#116163=DIRECTION('center_axis',(-1.0605752387249E-16,6.12323399573689E-17,
1.));
#116164=DIRECTION('ref_axis',(0.866025403784433,-0.50000000000001,1.22464679914735E-16));
#116165=DIRECTION('center_axis',(-0.866025403784445,-0.499999999999989,
0.));
#116166=DIRECTION('ref_axis',(-0.499999999999989,0.866025403784445,0.));
#116167=DIRECTION('center_axis',(-6.12323399573663E-17,1.06057523872491E-16,
1.));
#116168=DIRECTION('ref_axis',(0.499999999999989,-0.866025403784445,1.22464679914735E-16));
#116169=DIRECTION('center_axis',(0.,0.,1.));
#116170=DIRECTION('ref_axis',(1.,0.,0.));
#116171=DIRECTION('center_axis',(0.,0.,1.));
#116172=DIRECTION('ref_axis',(1.,0.,0.));
#116173=DIRECTION('',(0.,0.,-1.));
#116174=DIRECTION('center_axis',(0.,0.,1.));
#116175=DIRECTION('ref_axis',(1.,0.,0.));
#116176=DIRECTION('center_axis',(0.,0.,1.));
#116177=DIRECTION('ref_axis',(1.,0.,0.));
#116178=DIRECTION('center_axis',(0.,0.,1.));
#116179=DIRECTION('ref_axis',(1.,0.,0.));
#116180=DIRECTION('',(0.,0.,1.));
#116181=DIRECTION('center_axis',(0.,0.,1.));
#116182=DIRECTION('ref_axis',(1.,0.,0.));
#116183=DIRECTION('center_axis',(0.,0.,-1.));
#116184=DIRECTION('ref_axis',(-1.,0.,0.));
#116185=DIRECTION('center_axis',(0.,0.,1.));
#116186=DIRECTION('ref_axis',(1.,0.,0.));
#116187=DIRECTION('center_axis',(0.,0.,1.));
#116188=DIRECTION('ref_axis',(1.,0.,0.));
#116189=DIRECTION('center_axis',(0.,0.,1.));
#116190=DIRECTION('ref_axis',(1.,0.,0.));
#116191=DIRECTION('',(0.,0.,-1.));
#116192=DIRECTION('center_axis',(0.,0.,1.));
#116193=DIRECTION('ref_axis',(1.,0.,0.));
#116194=DIRECTION('center_axis',(0.,0.,1.));
#116195=DIRECTION('ref_axis',(1.,0.,0.));
#116196=DIRECTION('center_axis',(0.,0.,1.));
#116197=DIRECTION('ref_axis',(1.,0.,0.));
#116198=DIRECTION('',(0.,0.,1.));
#116199=DIRECTION('center_axis',(0.,0.,1.));
#116200=DIRECTION('ref_axis',(1.,0.,0.));
#116201=DIRECTION('center_axis',(0.,0.,1.));
#116202=DIRECTION('ref_axis',(1.,0.,0.));
#116203=DIRECTION('center_axis',(0.,0.,-1.));
#116204=DIRECTION('ref_axis',(-1.,0.,0.));
#366184=CARTESIAN_POINT('',(0.,0.,0.));
#366185=CARTESIAN_POINT('Origin',(0.,0.,1.25));
#366186=CARTESIAN_POINT('',(-2.40384615384615,-2.94386249795037E-16,0.555555555555555));
#366187=CARTESIAN_POINT('Origin',(0.,0.,0.555555555555555));
#366188=CARTESIAN_POINT('',(-2.40384615384615,-2.94386249795037E-16,1.25));
#366189=CARTESIAN_POINT('',(-2.40384615384615,-2.94386249795037E-16,1.25));
#366190=CARTESIAN_POINT('Origin',(0.,0.,1.25));
#366191=CARTESIAN_POINT('Origin',(0.,0.,-3.36777869765522E-16));
#366192=CARTESIAN_POINT('',(-2.40384615384615,-2.94386249795037E-16,-0.555555555555556));
#366193=CARTESIAN_POINT('Origin',(0.,0.,-0.555555555555556));
#366194=CARTESIAN_POINT('Origin',(-2.25,-2.75545529808155E-16,-3.36777869765522E-16));
#366195=CARTESIAN_POINT('Origin',(0.,0.,1.25));
#366196=CARTESIAN_POINT('',(-2.40384615384615,-2.94386249795037E-16,-1.25));
#366197=CARTESIAN_POINT('Origin',(0.,0.,-1.25));
#366198=CARTESIAN_POINT('',(-2.40384615384615,-2.94386249795037E-16,1.25));
#366199=CARTESIAN_POINT('Origin',(0.,0.,-1.25));
#366200=CARTESIAN_POINT('',(-3.,-3.67394039744206E-16,-1.125));
#366201=CARTESIAN_POINT('Origin',(0.,0.,-1.125));
#366202=CARTESIAN_POINT('',(-2.875,-3.52085954754864E-16,-1.25));
#366203=CARTESIAN_POINT('',(-2.875,-3.52085954754864E-16,-1.25));
#366204=CARTESIAN_POINT('Origin',(0.,0.,-1.25));
#366205=CARTESIAN_POINT('Origin',(0.,0.,1.25));
#366206=CARTESIAN_POINT('',(3.,3.67394039744206E-16,1.125));
#366207=CARTESIAN_POINT('',(-3.,-3.67394039744206E-16,1.125));
#366208=CARTESIAN_POINT('Origin',(0.,0.,1.125));
#366209=CARTESIAN_POINT('Origin',(0.,0.,1.125));
#366210=CARTESIAN_POINT('',(-3.,-3.67394039744206E-16,1.25));
#366211=CARTESIAN_POINT('Origin',(0.,0.,1.125));
#366212=CARTESIAN_POINT('',(2.875,-3.52085954754864E-16,1.25));
#366213=CARTESIAN_POINT('',(3.,-3.67394039744206E-16,1.125));
#366214=CARTESIAN_POINT('Origin',(0.,0.,1.25));
#366215=CARTESIAN_POINT('Origin',(0.,2.875,-1.25));
#366216=CARTESIAN_POINT('Origin',(0.,2.875,1.25));
#366217=CARTESIAN_POINT('Origin',(0.,0.,-9.75781955236954E-16));
#366218=CARTESIAN_POINT('',(-2.09615384615385,2.56704809821272E-16,0.555555555555555));
#366219=CARTESIAN_POINT('Origin',(0.,0.,0.555555555555555));
#366220=CARTESIAN_POINT('',(-2.09615384615385,-2.56704809821272E-16,-0.555555555555556));
#366221=CARTESIAN_POINT('Origin',(-2.25,-2.75545529808154E-16,-9.75781955236954E-16));
#366222=CARTESIAN_POINT('Origin',(0.,0.,-0.555555555555556));
#366223=CARTESIAN_POINT('Origin',(0.,0.,1.25));
#366224=CARTESIAN_POINT('',(-1.5,-1.83697019872103E-16,1.125));
#366225=CARTESIAN_POINT('Origin',(0.,0.,1.125));
#366226=CARTESIAN_POINT('',(-1.625,-1.99005104861445E-16,1.25));
#366227=CARTESIAN_POINT('',(-1.625,-1.99005104861445E-16,1.25));
#366228=CARTESIAN_POINT('Origin',(0.,0.,1.25));
#366229=CARTESIAN_POINT('Origin',(0.,0.,1.25));
#366230=CARTESIAN_POINT('',(1.5,1.91351062366774E-16,-1.125));
#366231=CARTESIAN_POINT('',(-1.5,-1.83697019872103E-16,-1.125));
#366232=CARTESIAN_POINT('Origin',(0.,0.,-1.125));
#366233=CARTESIAN_POINT('Origin',(0.,0.,-1.125));
#366234=CARTESIAN_POINT('',(-1.5,-1.83697019872103E-16,1.25));
#366235=CARTESIAN_POINT('Origin',(0.,0.,-1.125));
#366236=CARTESIAN_POINT('',(1.625,-1.99005104861445E-16,-1.25));
#366237=CARTESIAN_POINT('',(1.5,-1.83697019872103E-16,-1.125));
#366238=CARTESIAN_POINT('Origin',(0.,0.,-1.25));
#366239=CARTESIAN_POINT('Origin',(0.,0.,1.25));
#366240=CARTESIAN_POINT('',(-2.09615384615385,-2.56704809821272E-16,-1.25));
#366241=CARTESIAN_POINT('',(-2.09615384615385,-2.56704809821272E-16,1.25));
#366242=CARTESIAN_POINT('Origin',(0.,0.,-1.25));
#366243=CARTESIAN_POINT('Origin',(0.,0.,1.25));
#366244=CARTESIAN_POINT('',(-2.09615384615385,-2.56704809821272E-16,1.25));
#366245=CARTESIAN_POINT('Origin',(0.,0.,1.25));
#366246=CARTESIAN_POINT('',(-2.09615384615385,-2.56704809821272E-16,1.25));
#366247=CARTESIAN_POINT('Origin',(0.,2.09615384615385,1.25));
#366248=CARTESIAN_POINT('Origin',(0.,1.625,-1.25));
#366249=CARTESIAN_POINT('Origin',(0.,2.25,-3.36777869765522E-16));
#366250=CARTESIAN_POINT('',(-0.576463888168111,2.25,-3.36777869765522E-16));
#366251=CARTESIAN_POINT('',(0.576463888168111,2.25,-3.36777869765522E-16));
#366252=CARTESIAN_POINT('Origin',(0.,2.25,-3.36777869765522E-16));
#366253=CARTESIAN_POINT('Origin',(1.125,1.94855715851499,-3.36777869765522E-16));
#366254=CARTESIAN_POINT('',(0.625767628482067,2.23678910259904,-3.36777869765522E-16));
#366255=CARTESIAN_POINT('',(1.62423237151794,1.66032521443093,-3.36777869765522E-16));
#366256=CARTESIAN_POINT('Origin',(1.125,1.94855715851499,-3.36777869765522E-16));
#366257=CARTESIAN_POINT('Origin',(1.94855715851499,1.125,-3.36777869765522E-16));
#366258=CARTESIAN_POINT('',(1.66032521443094,1.62423237151793,-3.36777869765522E-16));
#366259=CARTESIAN_POINT('',(2.23678910259904,0.625767628482059,-3.36777869765522E-16));
#366260=CARTESIAN_POINT('Origin',(1.94855715851499,1.125,-3.36777869765522E-16));
#366261=CARTESIAN_POINT('Origin',(2.25,-7.85583301239705E-15,-3.36777869765522E-16));
#366262=CARTESIAN_POINT('',(2.25,0.576463888168103,-3.36777869765522E-16));
#366263=CARTESIAN_POINT('',(2.25,-0.576463888168119,-3.36777869765522E-16));
#366264=CARTESIAN_POINT('Origin',(2.25,-7.85583301239705E-15,-3.36777869765522E-16));
#366265=CARTESIAN_POINT('Origin',(1.94855715851498,-1.12500000000001,-3.36777869765522E-16));
#366266=CARTESIAN_POINT('',(2.23678910259904,-0.625767628482075,-3.36777869765522E-16));
#366267=CARTESIAN_POINT('',(1.66032521443092,-1.62423237151794,-3.36777869765522E-16));
#366268=CARTESIAN_POINT('Origin',(1.94855715851498,-1.12500000000001,-3.36777869765522E-16));
#366269=CARTESIAN_POINT('Origin',(1.12499999999999,-1.94855715851499,-3.36777869765522E-16));
#366270=CARTESIAN_POINT('',(1.62423237151793,-1.66032521443094,-3.36777869765522E-16));
#366271=CARTESIAN_POINT('',(0.625767628482051,-2.23678910259905,-3.36777869765522E-16));
#366272=CARTESIAN_POINT('Origin',(1.12499999999999,-1.94855715851499,-3.36777869765522E-16));
#366273=CARTESIAN_POINT('Origin',(-1.57116660247941E-14,-2.25,-3.36777869765522E-16));
#366274=CARTESIAN_POINT('',(0.576463888168095,-2.25,-3.36777869765522E-16));
#366275=CARTESIAN_POINT('',(-0.576463888168127,-2.25,-3.36777869765522E-16));
#366276=CARTESIAN_POINT('Origin',(-1.57116660247941E-14,-2.25,-3.36777869765522E-16));
#366277=CARTESIAN_POINT('Origin',(-1.12500000000002,-1.94855715851498,-3.36777869765522E-16));
#366278=CARTESIAN_POINT('',(-0.625767628482083,-2.23678910259904,-3.36777869765522E-16));
#366279=CARTESIAN_POINT('',(-1.62423237151795,-1.66032521443092,-3.36777869765522E-16));
#366280=CARTESIAN_POINT('Origin',(-1.12500000000002,-1.94855715851498,-3.36777869765522E-16));
#366281=CARTESIAN_POINT('Origin',(-1.948557158515,-1.12499999999998,-3.36777869765522E-16));
#366282=CARTESIAN_POINT('',(-1.66032521443095,-1.62423237151792,-3.36777869765522E-16));
#366283=CARTESIAN_POINT('',(-2.23678910259905,-0.625767628482044,-3.36777869765522E-16));
#366284=CARTESIAN_POINT('Origin',(-1.948557158515,-1.12499999999998,-3.36777869765522E-16));
#366285=CARTESIAN_POINT('Origin',(-2.25,2.35674990371912E-14,-3.36777869765522E-16));
#366286=CARTESIAN_POINT('',(-2.25000000000001,-0.576463888168087,-3.36777869765522E-16));
#366287=CARTESIAN_POINT('',(-2.24999999999999,0.576463888168134,-3.36777869765522E-16));
#366288=CARTESIAN_POINT('Origin',(-2.25,2.35674990371912E-14,-3.36777869765522E-16));
#366289=CARTESIAN_POINT('Origin',(-1.94855715851497,1.12500000000002,-3.36777869765522E-16));
#366290=CARTESIAN_POINT('',(-2.23678910259904,0.62576762848209,-3.36777869765522E-16));
#366291=CARTESIAN_POINT('',(-1.66032521443091,1.62423237151796,-3.36777869765522E-16));
#366292=CARTESIAN_POINT('Origin',(-1.94855715851497,1.12500000000002,-3.36777869765522E-16));
#366293=CARTESIAN_POINT('Origin',(-1.12499999999998,1.948557158515,-3.36777869765522E-16));
#366294=CARTESIAN_POINT('',(-1.62423237151791,1.66032521443095,-3.36777869765522E-16));
#366295=CARTESIAN_POINT('',(-0.625767628482036,2.23678910259905,-3.36777869765522E-16));
#366296=CARTESIAN_POINT('Origin',(-1.12499999999998,1.948557158515,-3.36777869765522E-16));
#366297=CARTESIAN_POINT('Origin',(0.,0.,1.25));
#366298=CARTESIAN_POINT('',(-2.40384615384615,-2.94386249795037E-16,1.1875));
#366299=CARTESIAN_POINT('Origin',(0.,0.,1.1875));
#366300=CARTESIAN_POINT('',(-2.40384615384615,-2.94386249795037E-16,0.576463888168111));
#366301=CARTESIAN_POINT('',(-2.40384615384615,-2.94386249795037E-16,1.25));
#366302=CARTESIAN_POINT('Origin',(0.,0.,0.576463888168111));
#366303=CARTESIAN_POINT('Origin',(0.,0.,1.25));
#366304=CARTESIAN_POINT('',(-2.09615384615385,-2.56704809821272E-16,0.576463888168111));
#366305=CARTESIAN_POINT('Origin',(0.,0.,0.576463888168111));
#366306=CARTESIAN_POINT('',(-2.09615384615385,-2.56704809821272E-16,1.1875));
#366307=CARTESIAN_POINT('',(-2.09615384615385,-2.56704809821272E-16,1.25));
#366308=CARTESIAN_POINT('Origin',(0.,0.,1.1875));
#366309=CARTESIAN_POINT('Origin',(0.,2.40384615384615,1.1875));
#366310=CARTESIAN_POINT('Origin',(0.,2.40384615384615,0.576463888168111));
#366311=CARTESIAN_POINT('Origin',(0.,0.,1.25));
#366312=CARTESIAN_POINT('',(-2.40384615384615,-2.94386249795037E-16,-0.576463888168111));
#366313=CARTESIAN_POINT('Origin',(0.,0.,-0.576463888168111));
#366314=CARTESIAN_POINT('',(-2.40384615384615,-2.94386249795037E-16,-1.1875));
#366315=CARTESIAN_POINT('',(-2.40384615384615,-2.94386249795037E-16,1.25));
#366316=CARTESIAN_POINT('Origin',(0.,0.,-1.1875));
#366317=CARTESIAN_POINT('Origin',(0.,0.,1.25));
#366318=CARTESIAN_POINT('',(-2.09615384615385,-2.56704809821272E-16,-1.1875));
#366319=CARTESIAN_POINT('Origin',(0.,0.,-1.1875));
#366320=CARTESIAN_POINT('',(-2.09615384615385,-2.56704809821272E-16,-0.576463888168111));
#366321=CARTESIAN_POINT('',(-2.09615384615385,-2.56704809821272E-16,1.25));
#366322=CARTESIAN_POINT('Origin',(0.,0.,-0.576463888168111));
#366323=CARTESIAN_POINT('Origin',(0.,2.40384615384615,-1.1875));
#366324=CARTESIAN_POINT('Origin',(0.,2.40384615384615,-0.576463888168111));
#459205=UNCERTAINTY_MEASURE_WITH_UNIT(LENGTH_MEASURE(0.01),#459243,
'DISTANCE_ACCURACY_VALUE',
'Maximum model space distance between geometric entities at asserted c
onnectivities');
#459216=UNCERTAINTY_MEASURE_WITH_UNIT(LENGTH_MEASURE(0.01),#459243,
'DISTANCE_ACCURACY_VALUE',
'Maximum model space distance between geometric entities at asserted c
onnectivities');
#459231=(
GEOMETRIC_REPRESENTATION_CONTEXT(3)
GLOBAL_UNCERTAINTY_ASSIGNED_CONTEXT((#459205))
GLOBAL_UNIT_ASSIGNED_CONTEXT((#459243,#459245,#459246))
REPRESENTATION_CONTEXT('','3D')
);
#459242=(
GEOMETRIC_REPRESENTATION_CONTEXT(3)
GLOBAL_UNCERTAINTY_ASSIGNED_CONTEXT((#459216))
GLOBAL_UNIT_ASSIGNED_CONTEXT((#459243,#459245,#459246))
REPRESENTATION_CONTEXT('','3D')
);
#459243=(
LENGTH_UNIT()
NAMED_UNIT(*)
SI_UNIT(.MILLI.,.METRE.)
);
#459245=(
NAMED_UNIT(*)
PLANE_ANGLE_UNIT()
SI_UNIT($,.RADIAN.)
);
#459246=(
NAMED_UNIT(*)
SI_UNIT($,.STERADIAN.)
SOLID_ANGLE_UNIT()
);
#459261=SHAPE_DEFINITION_REPRESENTATION(#459288,#459342);
#459288=PRODUCT_DEFINITION_SHAPE('',$,#459368);
#459342=SHAPE_REPRESENTATION('',(#99171),#459231);
#459353=PRODUCT_DEFINITION_CONTEXT('part definition',#459430,'design');
#459368=PRODUCT_DEFINITION('Shaft Ball Bearing','Shaft Ball Bearing',#459393,
#459353);
#459393=PRODUCT_DEFINITION_FORMATION('',$,#459446);
#459430=APPLICATION_CONTEXT(
'Core Data for Automotive Mechanical Design Process');
#459431=PRODUCT_CONTEXT('part definition',#459430,'mechanical');
#459446=PRODUCT('Shaft Ball Bearing','Shaft Ball Bearing',$,(#459431));
#459520=COLOUR_RGB('Grey',0.48,0.52,0.57);
#459521=FILL_AREA_STYLE_COLOUR('',#459520);
#459522=FILL_AREA_STYLE('',(#459521));
#459523=SURFACE_STYLE_FILL_AREA(#459522);
#459524=SURFACE_SIDE_STYLE('',(#459523));
#459525=SURFACE_STYLE_USAGE(.BOTH.,#459524);
#459526=PRESENTATION_STYLE_ASSIGNMENT((#459525));
ENDSEC;
END-ISO-10303-21;
